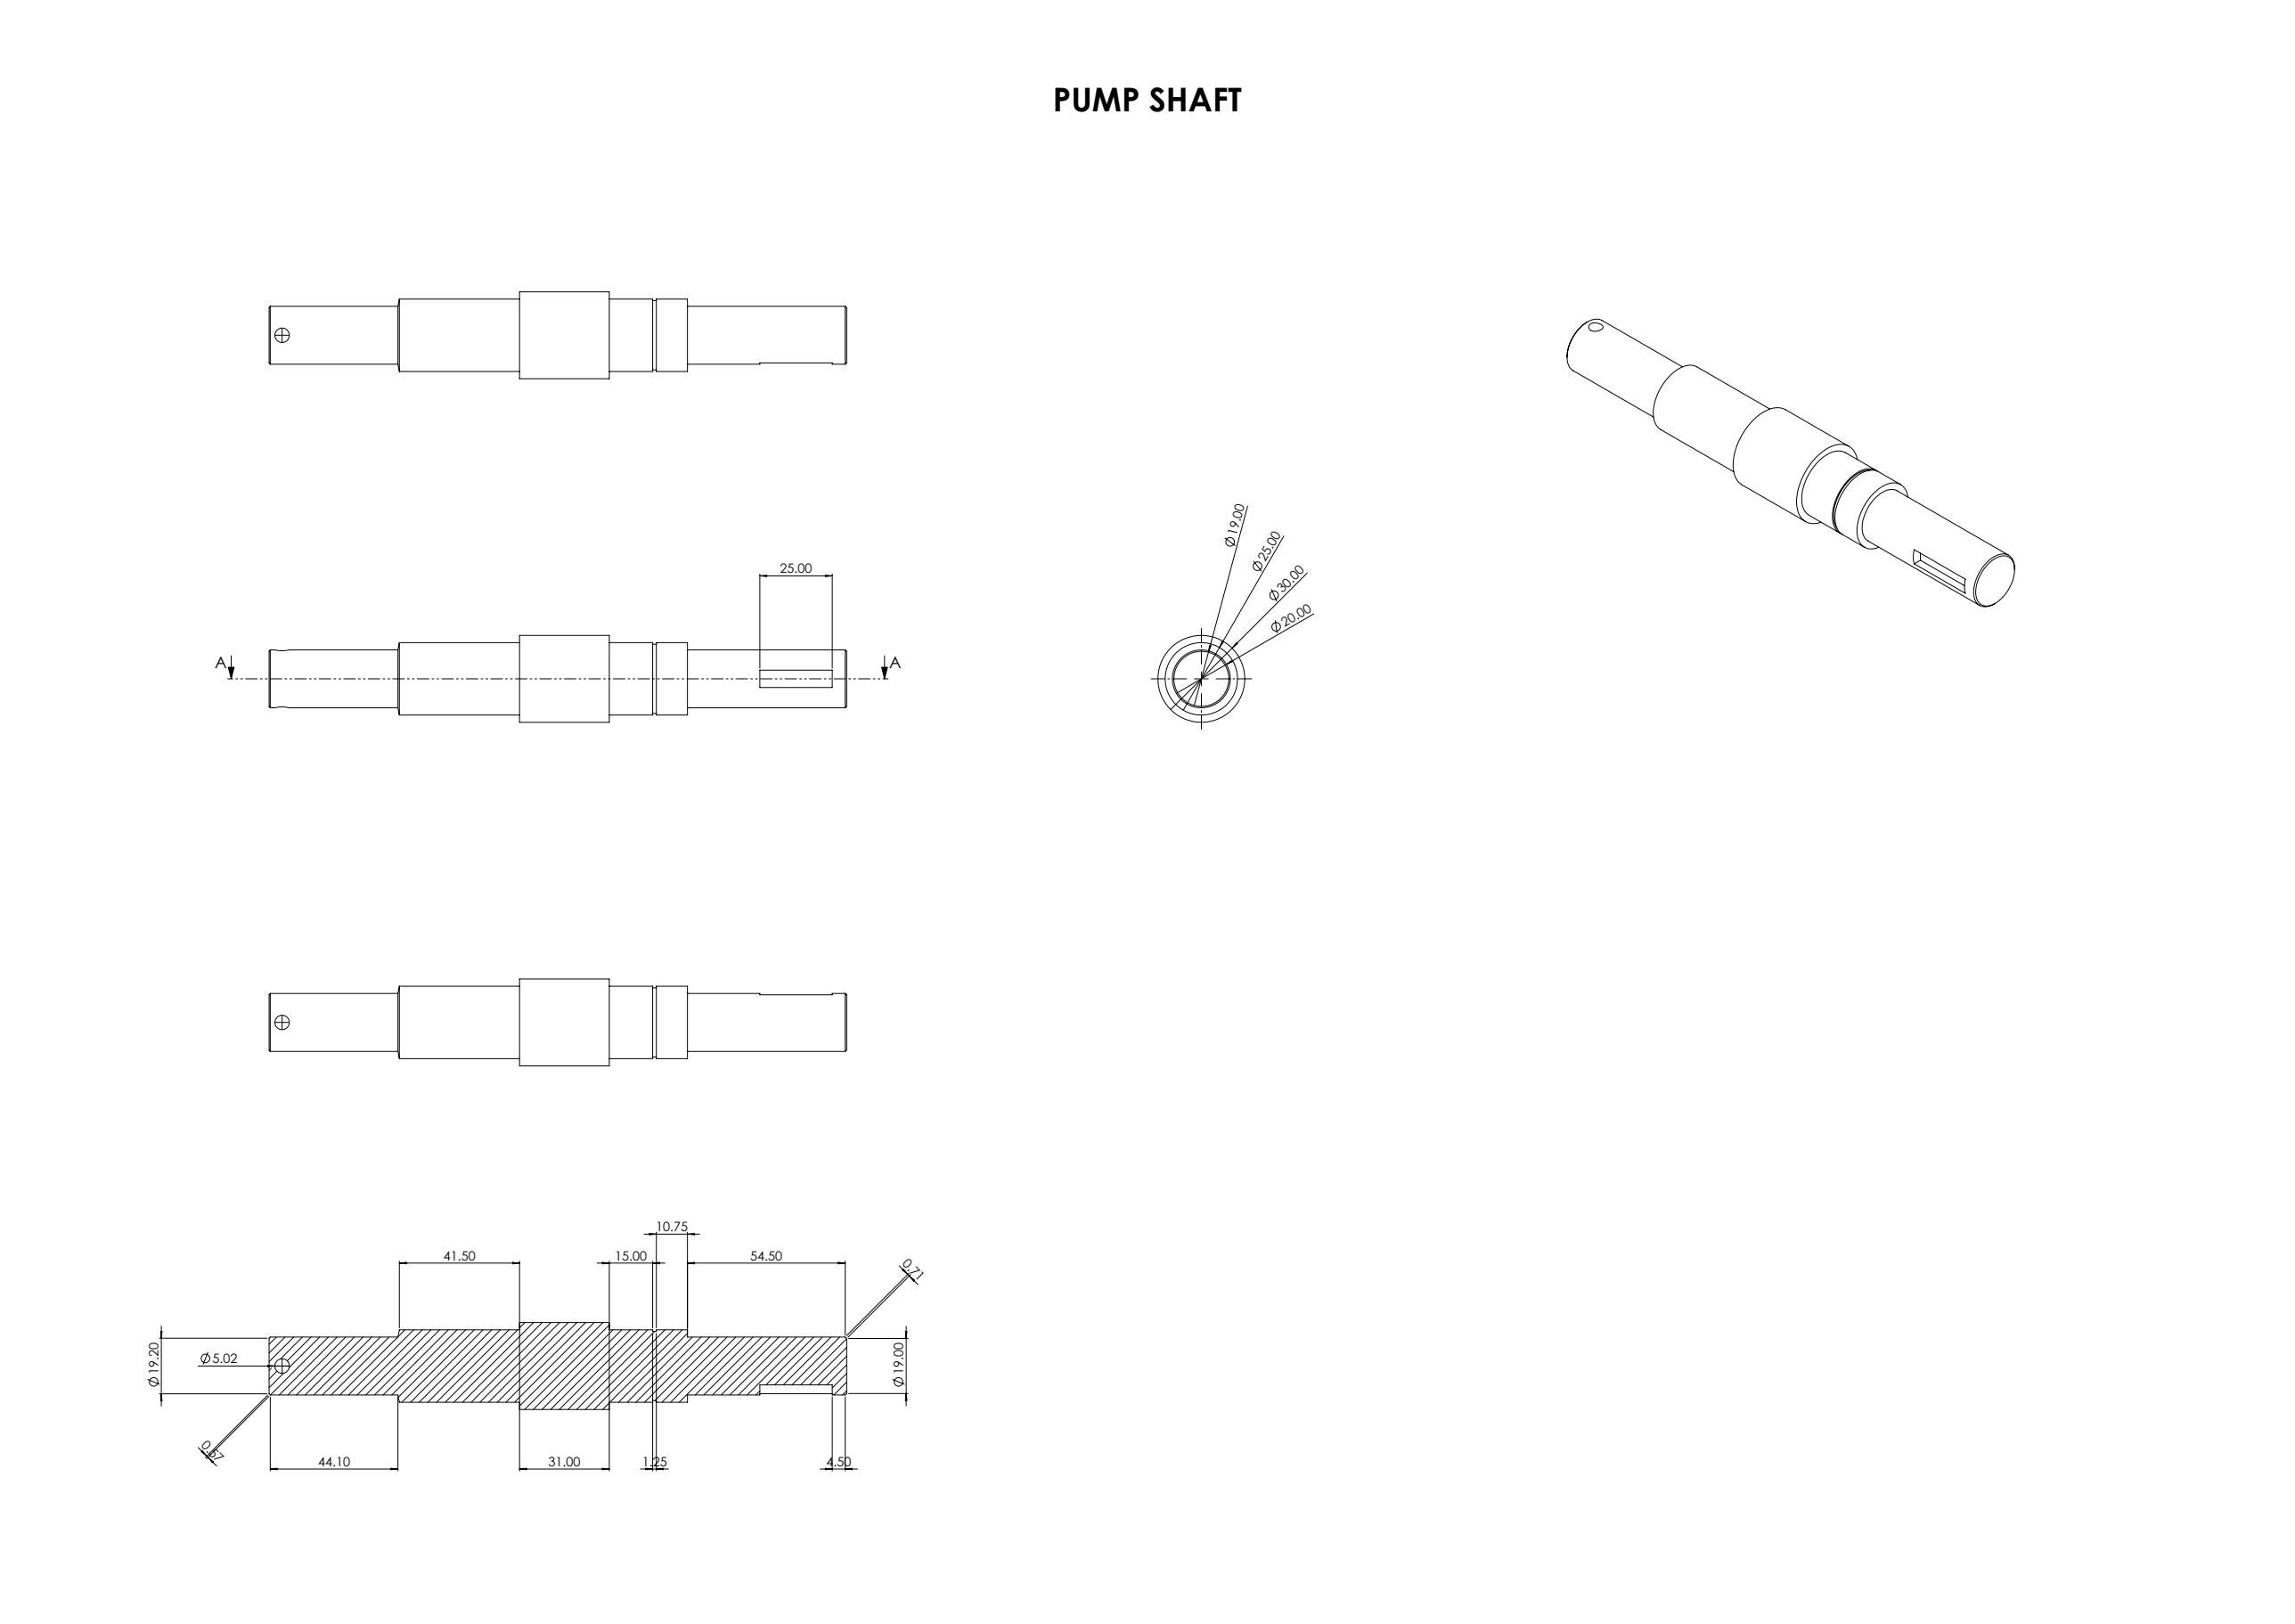
ISO-10303-21;
HEADER;
/* Generated by software containing ST-Developer
 * from STEP Tools, Inc. (www.steptools.com) 
 */

FILE_DESCRIPTION(
/* description */ (''),
/* implementation_level */ '2;1');

FILE_NAME(
/* name */ '05_Pump_Shaft.step',
/* time_stamp */ '2026-10-26T04:15:57-07:00',
/* author */ (''),
/* organization */ (''),
/* preprocessor_version */ 'ST-DEVELOPER v20.2',
/* originating_system */ 'Autodesk Translation Framework v15.15.0.0',
/* authorisation */ '');

FILE_SCHEMA (('AUTOMOTIVE_DESIGN { 1 0 10303 214 3 1 1 }'));
ENDSEC;

DATA;
#10=MECHANICAL_DESIGN_GEOMETRIC_PRESENTATION_REPRESENTATION('',(#456),#55737);
#363=CONICAL_SURFACE('',#29080,9.8,0.785398163397448);
#364=CONICAL_SURFACE('',#29084,11.25,1.37340076694502);
#365=CONICAL_SURFACE('',#29108,9.75,0.785398163397442);
#416=SHAPE_REPRESENTATION_RELATIONSHIP('SRR','None',#55825,#436);
#436=ADVANCED_BREP_SHAPE_REPRESENTATION('',(#476),#55721);
#456=STYLED_ITEM('',(#55991),#476);
#476=MANIFOLD_SOLID_BREP('Body1',#27225);
#683=FACE_BOUND('',#9449,.T.);
#684=FACE_BOUND('',#9453,.T.);
#685=FACE_BOUND('',#9456,.T.);
#686=FACE_BOUND('',#9459,.T.);
#687=FACE_BOUND('',#9462,.T.);
#688=FACE_BOUND('',#9465,.T.);
#689=FACE_BOUND('',#9467,.T.);
#1369=PLANE('',#29070);
#1370=PLANE('',#29072);
#1371=PLANE('',#29073);
#1372=PLANE('',#29074);
#1373=PLANE('',#29076);
#1374=PLANE('',#29078);
#1375=PLANE('',#29088);
#1376=PLANE('',#29092);
#1377=PLANE('',#29096);
#1378=PLANE('',#29100);
#1379=PLANE('',#29104);
#1380=PLANE('',#29110);
#3294=LINE('',#44964,#5665);
#3295=LINE('',#44966,#5666);
#3296=LINE('',#44967,#5667);
#3297=LINE('',#44970,#5668);
#3298=LINE('',#44972,#5669);
#3299=LINE('',#44973,#5670);
#3300=LINE('',#44976,#5671);
#3301=LINE('',#44978,#5672);
#3302=LINE('',#44979,#5673);
#3303=LINE('',#44982,#5674);
#3304=LINE('',#45009,#5675);
#3305=LINE('',#45071,#5676);
#3306=LINE('',#45075,#5677);
#3307=LINE('',#45076,#5678);
#3308=LINE('',#45080,#5679);
#3309=LINE('',#45084,#5680);
#3310=LINE('',#45091,#5681);
#3311=LINE('',#45098,#5682);
#3312=LINE('',#45105,#5683);
#3313=LINE('',#45112,#5684);
#3314=LINE('',#45119,#5685);
#3315=LINE('',#45123,#5686);
#5665=VECTOR('',#34732,10.);
#5666=VECTOR('',#34733,10.);
#5667=VECTOR('',#34734,10.);
#5668=VECTOR('',#34737,10.);
#5669=VECTOR('',#34738,10.);
#5670=VECTOR('',#34739,10.);
#5671=VECTOR('',#34742,10.);
#5672=VECTOR('',#34743,10.);
#5673=VECTOR('',#34744,10.);
#5674=VECTOR('',#34749,10.);
#5675=VECTOR('',#34754,2.51);
#5676=VECTOR('',#34763,9.8);
#5677=VECTOR('',#34768,10.);
#5678=VECTOR('',#34769,10.);
#5679=VECTOR('',#34774,11.25);
#5680=VECTOR('',#34779,12.5);
#5681=VECTOR('',#34788,15.);
#5682=VECTOR('',#34797,12.5);
#5683=VECTOR('',#34806,11.95);
#5684=VECTOR('',#34815,12.5);
#5685=VECTOR('',#34824,10.);
#5686=VECTOR('',#34829,9.75);
#6675=CYLINDRICAL_SURFACE('',#29077,2.51);
#6676=CYLINDRICAL_SURFACE('',#29082,10.);
#6677=CYLINDRICAL_SURFACE('',#29086,12.5);
#6678=CYLINDRICAL_SURFACE('',#29090,15.);
#6679=CYLINDRICAL_SURFACE('',#29094,12.5);
#6680=CYLINDRICAL_SURFACE('',#29098,11.95);
#6681=CYLINDRICAL_SURFACE('',#29102,12.5);
#6682=CYLINDRICAL_SURFACE('',#29106,10.);
#7792=FACE_OUTER_BOUND('',#9440,.T.);
#7793=FACE_OUTER_BOUND('',#9441,.T.);
#7794=FACE_OUTER_BOUND('',#9442,.T.);
#7795=FACE_OUTER_BOUND('',#9443,.T.);
#7796=FACE_OUTER_BOUND('',#9444,.T.);
#7797=FACE_OUTER_BOUND('',#9445,.T.);
#7798=FACE_OUTER_BOUND('',#9446,.T.);
#7799=FACE_OUTER_BOUND('',#9447,.T.);
#7800=FACE_OUTER_BOUND('',#9448,.T.);
#7801=FACE_OUTER_BOUND('',#9450,.T.);
#7802=FACE_OUTER_BOUND('',#9451,.T.);
#7803=FACE_OUTER_BOUND('',#9452,.T.);
#7804=FACE_OUTER_BOUND('',#9454,.T.);
#7805=FACE_OUTER_BOUND('',#9455,.T.);
#7806=FACE_OUTER_BOUND('',#9457,.T.);
#7807=FACE_OUTER_BOUND('',#9458,.T.);
#7808=FACE_OUTER_BOUND('',#9460,.T.);
#7809=FACE_OUTER_BOUND('',#9461,.T.);
#7810=FACE_OUTER_BOUND('',#9463,.T.);
#7811=FACE_OUTER_BOUND('',#9464,.T.);
#7812=FACE_OUTER_BOUND('',#9466,.T.);
#7813=FACE_OUTER_BOUND('',#9468,.T.);
#7814=FACE_OUTER_BOUND('',#9469,.T.);
#9440=EDGE_LOOP('',(#22784,#22785,#22786,#22787));
#9441=EDGE_LOOP('',(#22788,#22789,#22790,#22791));
#9442=EDGE_LOOP('',(#22792,#22793,#22794,#22795));
#9443=EDGE_LOOP('',(#22796,#22797,#22798,#22799));
#9444=EDGE_LOOP('',(#22800,#22801,#22802,#22803));
#9445=EDGE_LOOP('',(#22804,#22805,#22806,#22807,#22808,#22809,#22810));
#9446=EDGE_LOOP('',(#22811));
#9447=EDGE_LOOP('',(#22812,#22813,#22814,#22815));
#9448=EDGE_LOOP('',(#22816,#22817,#22818,#22819,#22820,#22821,#22822,#22823,
#22824));
#9449=EDGE_LOOP('',(#22825,#22826));
#9450=EDGE_LOOP('',(#22827,#22828,#22829,#22830));
#9451=EDGE_LOOP('',(#22831,#22832,#22833,#22834));
#9452=EDGE_LOOP('',(#22835));
#9453=EDGE_LOOP('',(#22836));
#9454=EDGE_LOOP('',(#22837,#22838,#22839,#22840));
#9455=EDGE_LOOP('',(#22841));
#9456=EDGE_LOOP('',(#22842));
#9457=EDGE_LOOP('',(#22843,#22844,#22845,#22846));
#9458=EDGE_LOOP('',(#22847));
#9459=EDGE_LOOP('',(#22848));
#9460=EDGE_LOOP('',(#22849,#22850,#22851,#22852));
#9461=EDGE_LOOP('',(#22853));
#9462=EDGE_LOOP('',(#22854));
#9463=EDGE_LOOP('',(#22855,#22856,#22857,#22858));
#9464=EDGE_LOOP('',(#22859));
#9465=EDGE_LOOP('',(#22860));
#9466=EDGE_LOOP('',(#22861,#22862,#22863,#22864));
#9467=EDGE_LOOP('',(#22865,#22866,#22867,#22868));
#9468=EDGE_LOOP('',(#22869,#22870,#22871,#22872));
#9469=EDGE_LOOP('',(#22873));
#10722=CIRCLE('',#29071,10.);
#10723=CIRCLE('',#29075,10.);
#10724=CIRCLE('',#29079,9.6);
#10725=CIRCLE('',#29081,10.);
#10726=CIRCLE('',#29083,10.);
#10727=CIRCLE('',#29085,12.5);
#10728=CIRCLE('',#29087,12.5);
#10729=CIRCLE('',#29089,15.);
#10730=CIRCLE('',#29091,15.);
#10731=CIRCLE('',#29093,12.5);
#10732=CIRCLE('',#29095,12.5);
#10733=CIRCLE('',#29097,11.95);
#10734=CIRCLE('',#29099,11.95);
#10735=CIRCLE('',#29101,12.5);
#10736=CIRCLE('',#29103,12.5);
#10737=CIRCLE('',#29105,10.);
#10738=CIRCLE('',#29107,10.);
#10739=CIRCLE('',#29109,9.5);
#11189=B_SPLINE_CURVE_WITH_KNOTS('',3,(#44987,#44988,#44989,#44990,#44991,
#44992,#44993,#44994,#44995,#44996),.UNSPECIFIED.,.F.,.F.,(4,2,2,2,4),(0.,
0.0949942193143224,0.189988438628645,0.284969155661888,0.379949872695131),
 .UNSPECIFIED.);
#11190=B_SPLINE_CURVE_WITH_KNOTS('',3,(#44998,#44999,#45000,#45001,#45002,
#45003,#45004,#45005,#45006,#45007),.UNSPECIFIED.,.F.,.F.,(4,2,2,2,4),(1.13984961808539,
1.23483033511864,1.32981105215188,1.4248052714662,1.51979949078052),
 .UNSPECIFIED.);
#11191=B_SPLINE_CURVE_WITH_KNOTS('',3,(#45011,#45012,#45013,#45014,#45015,
#45016,#45017,#45018,#45019,#45020),.UNSPECIFIED.,.F.,.F.,(4,2,2,2,4),(0.,
0.0949942193143224,0.189988438628645,0.284969155661888,0.379949872695131),
 .UNSPECIFIED.);
#11192=B_SPLINE_CURVE_WITH_KNOTS('',3,(#45021,#45022,#45023,#45024,#45025,
#45026,#45027,#45028,#45029,#45030,#45031,#45032,#45033,#45034,#45035,#45036,
#45037,#45038,#45039,#45040,#45041,#45042,#45043,#45044,#45045,#45046),
 .UNSPECIFIED.,.F.,.F.,(4,2,2,2,2,2,2,2,2,2,2,2,4),(0.379949872695131,0.474930589728375,
0.569911306761618,0.66490552607594,0.759899745390262,0.854893964704585,
0.949888184018907,1.04486890105215,1.13984961808539,1.23483033511864,1.32981105215188,
1.4248052714662,1.51979949078053),.UNSPECIFIED.);
#11193=B_SPLINE_CURVE_WITH_KNOTS('',3,(#45047,#45048,#45049,#45050,#45051,
#45052,#45053,#45054,#45055,#45056,#45057,#45058,#45059,#45060,#45061,#45062,
#45063,#45064),.UNSPECIFIED.,.F.,.F.,(4,2,2,2,2,2,2,2,4),(0.379949872695131,
0.474930589728374,0.569911306761618,0.66490552607594,0.759899745390262,
0.854893964704585,0.949888184018907,1.04486890105215,1.13984961808539),
 .UNSPECIFIED.);
#13022=VERTEX_POINT('',#44960);
#13023=VERTEX_POINT('',#44961);
#13024=VERTEX_POINT('',#44963);
#13025=VERTEX_POINT('',#44965);
#13026=VERTEX_POINT('',#44969);
#13027=VERTEX_POINT('',#44971);
#13028=VERTEX_POINT('',#44975);
#13029=VERTEX_POINT('',#44977);
#13030=VERTEX_POINT('',#44985);
#13031=VERTEX_POINT('',#44986);
#13032=VERTEX_POINT('',#44997);
#13033=VERTEX_POINT('',#45008);
#13034=VERTEX_POINT('',#45010);
#13035=VERTEX_POINT('',#45066);
#13036=VERTEX_POINT('',#45069);
#13037=VERTEX_POINT('',#45073);
#13038=VERTEX_POINT('',#45078);
#13039=VERTEX_POINT('',#45082);
#13040=VERTEX_POINT('',#45086);
#13041=VERTEX_POINT('',#45089);
#13042=VERTEX_POINT('',#45093);
#13043=VERTEX_POINT('',#45096);
#13044=VERTEX_POINT('',#45100);
#13045=VERTEX_POINT('',#45103);
#13046=VERTEX_POINT('',#45107);
#13047=VERTEX_POINT('',#45110);
#13048=VERTEX_POINT('',#45114);
#13049=VERTEX_POINT('',#45117);
#13050=VERTEX_POINT('',#45121);
#16396=EDGE_CURVE('',#13022,#13023,#10722,.T.);
#16397=EDGE_CURVE('',#13022,#13024,#3294,.T.);
#16398=EDGE_CURVE('',#13024,#13025,#3295,.T.);
#16399=EDGE_CURVE('',#13023,#13025,#3296,.T.);
#16400=EDGE_CURVE('',#13023,#13026,#3297,.T.);
#16401=EDGE_CURVE('',#13025,#13027,#3298,.T.);
#16402=EDGE_CURVE('',#13026,#13027,#3299,.T.);
#16403=EDGE_CURVE('',#13028,#13022,#3300,.T.);
#16404=EDGE_CURVE('',#13028,#13029,#3301,.T.);
#16405=EDGE_CURVE('',#13029,#13024,#3302,.T.);
#16406=EDGE_CURVE('',#13026,#13028,#10723,.T.);
#16407=EDGE_CURVE('',#13027,#13029,#3303,.T.);
#16408=EDGE_CURVE('',#13030,#13031,#11189,.T.);
#16409=EDGE_CURVE('',#13032,#13030,#11190,.T.);
#16410=EDGE_CURVE('',#13032,#13033,#3304,.T.);
#16411=EDGE_CURVE('',#13034,#13033,#11191,.T.);
#16412=EDGE_CURVE('',#13033,#13034,#11192,.T.);
#16413=EDGE_CURVE('',#13031,#13032,#11193,.T.);
#16414=EDGE_CURVE('',#13035,#13035,#10724,.T.);
#16415=EDGE_CURVE('',#13036,#13036,#10725,.T.);
#16416=EDGE_CURVE('',#13036,#13035,#3305,.T.);
#16417=EDGE_CURVE('',#13037,#13037,#10726,.T.);
#16418=EDGE_CURVE('',#13037,#13031,#3306,.T.);
#16419=EDGE_CURVE('',#13032,#13036,#3307,.T.);
#16420=EDGE_CURVE('',#13038,#13038,#10727,.T.);
#16421=EDGE_CURVE('',#13038,#13037,#3308,.T.);
#16422=EDGE_CURVE('',#13039,#13039,#10728,.T.);
#16423=EDGE_CURVE('',#13039,#13038,#3309,.T.);
#16424=EDGE_CURVE('',#13040,#13040,#10729,.T.);
#16425=EDGE_CURVE('',#13041,#13041,#10730,.T.);
#16426=EDGE_CURVE('',#13041,#13040,#3310,.T.);
#16427=EDGE_CURVE('',#13042,#13042,#10731,.T.);
#16428=EDGE_CURVE('',#13043,#13043,#10732,.T.);
#16429=EDGE_CURVE('',#13043,#13042,#3311,.T.);
#16430=EDGE_CURVE('',#13044,#13044,#10733,.T.);
#16431=EDGE_CURVE('',#13045,#13045,#10734,.T.);
#16432=EDGE_CURVE('',#13045,#13044,#3312,.T.);
#16433=EDGE_CURVE('',#13046,#13046,#10735,.T.);
#16434=EDGE_CURVE('',#13047,#13047,#10736,.T.);
#16435=EDGE_CURVE('',#13047,#13046,#3313,.T.);
#16436=EDGE_CURVE('',#13048,#13048,#10737,.T.);
#16437=EDGE_CURVE('',#13049,#13049,#10738,.T.);
#16438=EDGE_CURVE('',#13049,#13048,#3314,.T.);
#16439=EDGE_CURVE('',#13050,#13050,#10739,.T.);
#16440=EDGE_CURVE('',#13050,#13049,#3315,.T.);
#22784=ORIENTED_EDGE('',*,*,#16396,.F.);
#22785=ORIENTED_EDGE('',*,*,#16397,.T.);
#22786=ORIENTED_EDGE('',*,*,#16398,.T.);
#22787=ORIENTED_EDGE('',*,*,#16399,.F.);
#22788=ORIENTED_EDGE('',*,*,#16400,.F.);
#22789=ORIENTED_EDGE('',*,*,#16399,.T.);
#22790=ORIENTED_EDGE('',*,*,#16401,.T.);
#22791=ORIENTED_EDGE('',*,*,#16402,.F.);
#22792=ORIENTED_EDGE('',*,*,#16403,.F.);
#22793=ORIENTED_EDGE('',*,*,#16404,.T.);
#22794=ORIENTED_EDGE('',*,*,#16405,.T.);
#22795=ORIENTED_EDGE('',*,*,#16397,.F.);
#22796=ORIENTED_EDGE('',*,*,#16406,.F.);
#22797=ORIENTED_EDGE('',*,*,#16402,.T.);
#22798=ORIENTED_EDGE('',*,*,#16407,.T.);
#22799=ORIENTED_EDGE('',*,*,#16404,.F.);
#22800=ORIENTED_EDGE('',*,*,#16398,.F.);
#22801=ORIENTED_EDGE('',*,*,#16405,.F.);
#22802=ORIENTED_EDGE('',*,*,#16407,.F.);
#22803=ORIENTED_EDGE('',*,*,#16401,.F.);
#22804=ORIENTED_EDGE('',*,*,#16408,.F.);
#22805=ORIENTED_EDGE('',*,*,#16409,.F.);
#22806=ORIENTED_EDGE('',*,*,#16410,.T.);
#22807=ORIENTED_EDGE('',*,*,#16411,.F.);
#22808=ORIENTED_EDGE('',*,*,#16412,.F.);
#22809=ORIENTED_EDGE('',*,*,#16410,.F.);
#22810=ORIENTED_EDGE('',*,*,#16413,.F.);
#22811=ORIENTED_EDGE('',*,*,#16414,.F.);
#22812=ORIENTED_EDGE('',*,*,#16415,.F.);
#22813=ORIENTED_EDGE('',*,*,#16416,.T.);
#22814=ORIENTED_EDGE('',*,*,#16414,.T.);
#22815=ORIENTED_EDGE('',*,*,#16416,.F.);
#22816=ORIENTED_EDGE('',*,*,#16417,.F.);
#22817=ORIENTED_EDGE('',*,*,#16418,.T.);
#22818=ORIENTED_EDGE('',*,*,#16413,.T.);
#22819=ORIENTED_EDGE('',*,*,#16419,.T.);
#22820=ORIENTED_EDGE('',*,*,#16415,.T.);
#22821=ORIENTED_EDGE('',*,*,#16419,.F.);
#22822=ORIENTED_EDGE('',*,*,#16409,.T.);
#22823=ORIENTED_EDGE('',*,*,#16408,.T.);
#22824=ORIENTED_EDGE('',*,*,#16418,.F.);
#22825=ORIENTED_EDGE('',*,*,#16411,.T.);
#22826=ORIENTED_EDGE('',*,*,#16412,.T.);
#22827=ORIENTED_EDGE('',*,*,#16420,.F.);
#22828=ORIENTED_EDGE('',*,*,#16421,.T.);
#22829=ORIENTED_EDGE('',*,*,#16417,.T.);
#22830=ORIENTED_EDGE('',*,*,#16421,.F.);
#22831=ORIENTED_EDGE('',*,*,#16422,.F.);
#22832=ORIENTED_EDGE('',*,*,#16423,.T.);
#22833=ORIENTED_EDGE('',*,*,#16420,.T.);
#22834=ORIENTED_EDGE('',*,*,#16423,.F.);
#22835=ORIENTED_EDGE('',*,*,#16424,.F.);
#22836=ORIENTED_EDGE('',*,*,#16422,.T.);
#22837=ORIENTED_EDGE('',*,*,#16425,.F.);
#22838=ORIENTED_EDGE('',*,*,#16426,.T.);
#22839=ORIENTED_EDGE('',*,*,#16424,.T.);
#22840=ORIENTED_EDGE('',*,*,#16426,.F.);
#22841=ORIENTED_EDGE('',*,*,#16425,.T.);
#22842=ORIENTED_EDGE('',*,*,#16427,.F.);
#22843=ORIENTED_EDGE('',*,*,#16428,.F.);
#22844=ORIENTED_EDGE('',*,*,#16429,.T.);
#22845=ORIENTED_EDGE('',*,*,#16427,.T.);
#22846=ORIENTED_EDGE('',*,*,#16429,.F.);
#22847=ORIENTED_EDGE('',*,*,#16428,.T.);
#22848=ORIENTED_EDGE('',*,*,#16430,.F.);
#22849=ORIENTED_EDGE('',*,*,#16431,.F.);
#22850=ORIENTED_EDGE('',*,*,#16432,.T.);
#22851=ORIENTED_EDGE('',*,*,#16430,.T.);
#22852=ORIENTED_EDGE('',*,*,#16432,.F.);
#22853=ORIENTED_EDGE('',*,*,#16433,.F.);
#22854=ORIENTED_EDGE('',*,*,#16431,.T.);
#22855=ORIENTED_EDGE('',*,*,#16434,.F.);
#22856=ORIENTED_EDGE('',*,*,#16435,.T.);
#22857=ORIENTED_EDGE('',*,*,#16433,.T.);
#22858=ORIENTED_EDGE('',*,*,#16435,.F.);
#22859=ORIENTED_EDGE('',*,*,#16434,.T.);
#22860=ORIENTED_EDGE('',*,*,#16436,.F.);
#22861=ORIENTED_EDGE('',*,*,#16437,.F.);
#22862=ORIENTED_EDGE('',*,*,#16438,.T.);
#22863=ORIENTED_EDGE('',*,*,#16436,.T.);
#22864=ORIENTED_EDGE('',*,*,#16438,.F.);
#22865=ORIENTED_EDGE('',*,*,#16406,.T.);
#22866=ORIENTED_EDGE('',*,*,#16403,.T.);
#22867=ORIENTED_EDGE('',*,*,#16396,.T.);
#22868=ORIENTED_EDGE('',*,*,#16400,.T.);
#22869=ORIENTED_EDGE('',*,*,#16439,.F.);
#22870=ORIENTED_EDGE('',*,*,#16440,.T.);
#22871=ORIENTED_EDGE('',*,*,#16437,.T.);
#22872=ORIENTED_EDGE('',*,*,#16440,.F.);
#22873=ORIENTED_EDGE('',*,*,#16439,.T.);
#26616=ADVANCED_FACE('',(#7792),#1369,.F.);
#26617=ADVANCED_FACE('',(#7793),#1370,.F.);
#26618=ADVANCED_FACE('',(#7794),#1371,.F.);
#26619=ADVANCED_FACE('',(#7795),#1372,.F.);
#26620=ADVANCED_FACE('',(#7796),#1373,.F.);
#26621=ADVANCED_FACE('',(#7797),#6675,.F.);
#26622=ADVANCED_FACE('',(#7798),#1374,.T.);
#26623=ADVANCED_FACE('',(#7799),#363,.T.);
#26624=ADVANCED_FACE('',(#7800,#683),#6676,.T.);
#26625=ADVANCED_FACE('',(#7801),#364,.T.);
#26626=ADVANCED_FACE('',(#7802),#6677,.T.);
#26627=ADVANCED_FACE('',(#7803,#684),#1375,.T.);
#26628=ADVANCED_FACE('',(#7804),#6678,.T.);
#26629=ADVANCED_FACE('',(#7805,#685),#1376,.T.);
#26630=ADVANCED_FACE('',(#7806),#6679,.T.);
#26631=ADVANCED_FACE('',(#7807,#686),#1377,.T.);
#26632=ADVANCED_FACE('',(#7808),#6680,.T.);
#26633=ADVANCED_FACE('',(#7809,#687),#1378,.T.);
#26634=ADVANCED_FACE('',(#7810),#6681,.T.);
#26635=ADVANCED_FACE('',(#7811,#688),#1379,.T.);
#26636=ADVANCED_FACE('',(#7812,#689),#6682,.T.);
#26637=ADVANCED_FACE('',(#7813),#365,.T.);
#26638=ADVANCED_FACE('',(#7814),#1380,.T.);
#27225=CLOSED_SHELL('',(#26616,#26617,#26618,#26619,#26620,#26621,#26622,
#26623,#26624,#26625,#26626,#26627,#26628,#26629,#26630,#26631,#26632,#26633,
#26634,#26635,#26636,#26637,#26638));
#29069=AXIS2_PLACEMENT_3D('',#44958,#34726,#34727);
#29070=AXIS2_PLACEMENT_3D('',#44959,#34728,#34729);
#29071=AXIS2_PLACEMENT_3D('',#44962,#34730,#34731);
#29072=AXIS2_PLACEMENT_3D('',#44968,#34735,#34736);
#29073=AXIS2_PLACEMENT_3D('',#44974,#34740,#34741);
#29074=AXIS2_PLACEMENT_3D('',#44980,#34745,#34746);
#29075=AXIS2_PLACEMENT_3D('',#44981,#34747,#34748);
#29076=AXIS2_PLACEMENT_3D('',#44983,#34750,#34751);
#29077=AXIS2_PLACEMENT_3D('',#44984,#34752,#34753);
#29078=AXIS2_PLACEMENT_3D('',#45065,#34755,#34756);
#29079=AXIS2_PLACEMENT_3D('',#45067,#34757,#34758);
#29080=AXIS2_PLACEMENT_3D('',#45068,#34759,#34760);
#29081=AXIS2_PLACEMENT_3D('',#45070,#34761,#34762);
#29082=AXIS2_PLACEMENT_3D('',#45072,#34764,#34765);
#29083=AXIS2_PLACEMENT_3D('',#45074,#34766,#34767);
#29084=AXIS2_PLACEMENT_3D('',#45077,#34770,#34771);
#29085=AXIS2_PLACEMENT_3D('',#45079,#34772,#34773);
#29086=AXIS2_PLACEMENT_3D('',#45081,#34775,#34776);
#29087=AXIS2_PLACEMENT_3D('',#45083,#34777,#34778);
#29088=AXIS2_PLACEMENT_3D('',#45085,#34780,#34781);
#29089=AXIS2_PLACEMENT_3D('',#45087,#34782,#34783);
#29090=AXIS2_PLACEMENT_3D('',#45088,#34784,#34785);
#29091=AXIS2_PLACEMENT_3D('',#45090,#34786,#34787);
#29092=AXIS2_PLACEMENT_3D('',#45092,#34789,#34790);
#29093=AXIS2_PLACEMENT_3D('',#45094,#34791,#34792);
#29094=AXIS2_PLACEMENT_3D('',#45095,#34793,#34794);
#29095=AXIS2_PLACEMENT_3D('',#45097,#34795,#34796);
#29096=AXIS2_PLACEMENT_3D('',#45099,#34798,#34799);
#29097=AXIS2_PLACEMENT_3D('',#45101,#34800,#34801);
#29098=AXIS2_PLACEMENT_3D('',#45102,#34802,#34803);
#29099=AXIS2_PLACEMENT_3D('',#45104,#34804,#34805);
#29100=AXIS2_PLACEMENT_3D('',#45106,#34807,#34808);
#29101=AXIS2_PLACEMENT_3D('',#45108,#34809,#34810);
#29102=AXIS2_PLACEMENT_3D('',#45109,#34811,#34812);
#29103=AXIS2_PLACEMENT_3D('',#45111,#34813,#34814);
#29104=AXIS2_PLACEMENT_3D('',#45113,#34816,#34817);
#29105=AXIS2_PLACEMENT_3D('',#45115,#34818,#34819);
#29106=AXIS2_PLACEMENT_3D('',#45116,#34820,#34821);
#29107=AXIS2_PLACEMENT_3D('',#45118,#34822,#34823);
#29108=AXIS2_PLACEMENT_3D('',#45120,#34825,#34826);
#29109=AXIS2_PLACEMENT_3D('',#45122,#34827,#34828);
#29110=AXIS2_PLACEMENT_3D('',#45124,#34830,#34831);
#34726=DIRECTION('axis',(0.,0.,1.));
#34727=DIRECTION('refdir',(1.,0.,0.));
#34728=DIRECTION('center_axis',(-1.,0.,0.));
#34729=DIRECTION('ref_axis',(0.,1.,0.));
#34730=DIRECTION('center_axis',(-1.,0.,0.));
#34731=DIRECTION('ref_axis',(0.,1.,0.));
#34732=DIRECTION('',(0.,0.,-1.));
#34733=DIRECTION('',(0.,1.,0.));
#34734=DIRECTION('',(0.,0.,-1.));
#34735=DIRECTION('center_axis',(0.,1.,0.));
#34736=DIRECTION('ref_axis',(1.,0.,0.));
#34737=DIRECTION('',(1.,0.,0.));
#34738=DIRECTION('',(1.,0.,0.));
#34739=DIRECTION('',(0.,0.,-1.));
#34740=DIRECTION('center_axis',(0.,-1.,0.));
#34741=DIRECTION('ref_axis',(-1.,0.,0.));
#34742=DIRECTION('',(-1.,0.,0.));
#34743=DIRECTION('',(0.,0.,-1.));
#34744=DIRECTION('',(-1.,0.,0.));
#34745=DIRECTION('center_axis',(1.,0.,0.));
#34746=DIRECTION('ref_axis',(0.,-1.,0.));
#34747=DIRECTION('center_axis',(1.,0.,0.));
#34748=DIRECTION('ref_axis',(0.,1.,0.));
#34749=DIRECTION('',(0.,-1.,0.));
#34750=DIRECTION('center_axis',(0.,0.,-1.));
#34751=DIRECTION('ref_axis',(-1.,0.,0.));
#34752=DIRECTION('center_axis',(0.,1.,0.));
#34753=DIRECTION('ref_axis',(1.,0.,0.));
#34754=DIRECTION('',(0.,1.,0.));
#34755=DIRECTION('center_axis',(-1.,0.,0.));
#34756=DIRECTION('ref_axis',(0.,0.,1.));
#34757=DIRECTION('center_axis',(1.,0.,0.));
#34758=DIRECTION('ref_axis',(0.,0.,-1.));
#34759=DIRECTION('center_axis',(1.,0.,0.));
#34760=DIRECTION('ref_axis',(0.,1.,0.));
#34761=DIRECTION('center_axis',(1.,0.,0.));
#34762=DIRECTION('ref_axis',(0.,0.,-1.));
#34763=DIRECTION('',(-0.707106781186548,0.707106781186548,8.65956056235494E-17));
#34764=DIRECTION('center_axis',(1.,0.,0.));
#34765=DIRECTION('ref_axis',(0.,1.,0.));
#34766=DIRECTION('center_axis',(1.,0.,0.));
#34767=DIRECTION('ref_axis',(0.,0.,-1.));
#34768=DIRECTION('',(-1.,0.,0.));
#34769=DIRECTION('',(-1.,0.,0.));
#34770=DIRECTION('center_axis',(1.,0.,0.));
#34771=DIRECTION('ref_axis',(0.,1.,0.));
#34772=DIRECTION('center_axis',(1.,0.,0.));
#34773=DIRECTION('ref_axis',(0.,0.,-1.));
#34774=DIRECTION('',(-0.196116135138183,0.98058067569092,1.20086498579063E-16));
#34775=DIRECTION('center_axis',(1.,0.,0.));
#34776=DIRECTION('ref_axis',(0.,1.,0.));
#34777=DIRECTION('center_axis',(1.,0.,0.));
#34778=DIRECTION('ref_axis',(0.,0.,-1.));
#34779=DIRECTION('',(-1.,0.,0.));
#34780=DIRECTION('center_axis',(-1.,0.,0.));
#34781=DIRECTION('ref_axis',(0.,0.,1.));
#34782=DIRECTION('center_axis',(1.,0.,0.));
#34783=DIRECTION('ref_axis',(0.,0.,-1.));
#34784=DIRECTION('center_axis',(1.,0.,0.));
#34785=DIRECTION('ref_axis',(0.,1.,0.));
#34786=DIRECTION('center_axis',(1.,0.,0.));
#34787=DIRECTION('ref_axis',(0.,0.,-1.));
#34788=DIRECTION('',(-1.,0.,0.));
#34789=DIRECTION('center_axis',(1.,0.,0.));
#34790=DIRECTION('ref_axis',(0.,0.,-1.));
#34791=DIRECTION('center_axis',(1.,0.,0.));
#34792=DIRECTION('ref_axis',(0.,0.,-1.));
#34793=DIRECTION('center_axis',(1.,0.,0.));
#34794=DIRECTION('ref_axis',(0.,1.,0.));
#34795=DIRECTION('center_axis',(1.,0.,0.));
#34796=DIRECTION('ref_axis',(0.,0.,-1.));
#34797=DIRECTION('',(-1.,0.,0.));
#34798=DIRECTION('center_axis',(1.,0.,0.));
#34799=DIRECTION('ref_axis',(0.,0.,-1.));
#34800=DIRECTION('center_axis',(1.,0.,0.));
#34801=DIRECTION('ref_axis',(0.,0.,-1.));
#34802=DIRECTION('center_axis',(1.,0.,0.));
#34803=DIRECTION('ref_axis',(0.,1.,0.));
#34804=DIRECTION('center_axis',(1.,0.,0.));
#34805=DIRECTION('ref_axis',(0.,0.,-1.));
#34806=DIRECTION('',(-1.,0.,0.));
#34807=DIRECTION('center_axis',(-1.,0.,0.));
#34808=DIRECTION('ref_axis',(0.,0.,1.));
#34809=DIRECTION('center_axis',(1.,0.,0.));
#34810=DIRECTION('ref_axis',(0.,0.,-1.));
#34811=DIRECTION('center_axis',(1.,0.,0.));
#34812=DIRECTION('ref_axis',(0.,1.,0.));
#34813=DIRECTION('center_axis',(1.,0.,0.));
#34814=DIRECTION('ref_axis',(0.,0.,-1.));
#34815=DIRECTION('',(-1.,0.,0.));
#34816=DIRECTION('center_axis',(1.,0.,0.));
#34817=DIRECTION('ref_axis',(0.,0.,-1.));
#34818=DIRECTION('center_axis',(1.,0.,0.));
#34819=DIRECTION('ref_axis',(0.,0.,-1.));
#34820=DIRECTION('center_axis',(1.,0.,0.));
#34821=DIRECTION('ref_axis',(0.,1.,0.));
#34822=DIRECTION('center_axis',(1.,0.,0.));
#34823=DIRECTION('ref_axis',(0.,0.,-1.));
#34824=DIRECTION('',(-1.,0.,0.));
#34825=DIRECTION('center_axis',(-1.,0.,0.));
#34826=DIRECTION('ref_axis',(0.,1.,0.));
#34827=DIRECTION('center_axis',(1.,0.,0.));
#34828=DIRECTION('ref_axis',(0.,0.,-1.));
#34829=DIRECTION('',(-0.707106781186552,-0.707106781186543,-8.65956056235487E-17));
#34830=DIRECTION('center_axis',(1.,0.,0.));
#34831=DIRECTION('ref_axis',(0.,0.,-1.));
#44958=CARTESIAN_POINT('',(0.,0.,0.));
#44959=CARTESIAN_POINT('Origin',(165.,-3.,10.));
#44960=CARTESIAN_POINT('',(165.,-3.,9.53939201416946));
#44961=CARTESIAN_POINT('',(165.,3.,9.53939201416946));
#44962=CARTESIAN_POINT('Origin',(165.,0.,0.));
#44963=CARTESIAN_POINT('',(165.,-3.,6.5));
#44964=CARTESIAN_POINT('',(165.,-3.,10.));
#44965=CARTESIAN_POINT('',(165.,3.,6.5));
#44966=CARTESIAN_POINT('',(165.,3.,6.5));
#44967=CARTESIAN_POINT('',(165.,3.,10.));
#44968=CARTESIAN_POINT('Origin',(165.,3.,10.));
#44969=CARTESIAN_POINT('',(190.,3.,9.53939201416946));
#44970=CARTESIAN_POINT('',(167.25,3.,9.53939201416946));
#44971=CARTESIAN_POINT('',(190.,3.,6.5));
#44972=CARTESIAN_POINT('',(190.,3.,6.5));
#44973=CARTESIAN_POINT('',(190.,3.,10.));
#44974=CARTESIAN_POINT('Origin',(190.,-3.,10.));
#44975=CARTESIAN_POINT('',(190.,-3.,9.53939201416946));
#44976=CARTESIAN_POINT('',(167.25,-3.,9.53939201416946));
#44977=CARTESIAN_POINT('',(190.,-3.,6.5));
#44978=CARTESIAN_POINT('',(190.,-3.,10.));
#44979=CARTESIAN_POINT('',(165.,-3.,6.5));
#44980=CARTESIAN_POINT('Origin',(190.,3.,10.));
#44981=CARTESIAN_POINT('Origin',(190.,0.,0.));
#44982=CARTESIAN_POINT('',(190.,-3.,6.5));
#44983=CARTESIAN_POINT('Origin',(177.5,0.,6.5));
#44984=CARTESIAN_POINT('Origin',(0.,-11.,0.));
#44985=CARTESIAN_POINT('',(1.38777878078145E-16,-9.67987086690727,2.51));
#44986=CARTESIAN_POINT('',(2.51,-10.,-6.81712338612749E-16));
#44987=CARTESIAN_POINT('Ctrl Pts',(-6.93889390390723E-17,-9.67987086690727,
2.51));
#44988=CARTESIAN_POINT('Ctrl Pts',(0.316647397714408,-9.67987086690727,
2.51));
#44989=CARTESIAN_POINT('Ctrl Pts',(0.653424667393654,-9.69702654534655,
2.4464396819459));
#44990=CARTESIAN_POINT('Ctrl Pts',(1.27140541887387,-9.75816738483577,2.18987665098482));
#44991=CARTESIAN_POINT('Ctrl Pts',(1.55273320805174,-9.80118127300772,1.99694283350472));
#44992=CARTESIAN_POINT('Ctrl Pts',(1.99691126398784,-9.8812874714592,1.55276477756863));
#44993=CARTESIAN_POINT('Ctrl Pts',(2.18986969302056,-9.92370211108617,1.27142384596148));
#44994=CARTESIAN_POINT('Ctrl Pts',(2.44645069525432,-9.98345908137755,0.653396472215422));
#44995=CARTESIAN_POINT('Ctrl Pts',(2.51,-10.,0.316602390110811));
#44996=CARTESIAN_POINT('Ctrl Pts',(2.51,-10.,-6.93889390390723E-17));
#44997=CARTESIAN_POINT('',(-2.51,-10.,3.07386346585986E-16));
#44998=CARTESIAN_POINT('Ctrl Pts',(-2.51,-10.,-4.16333634234434E-16));
#44999=CARTESIAN_POINT('Ctrl Pts',(-2.51,-10.,0.31660239011081));
#45000=CARTESIAN_POINT('Ctrl Pts',(-2.44645069525432,-9.98345908137755,
0.65339647221542));
#45001=CARTESIAN_POINT('Ctrl Pts',(-2.18986969302057,-9.92370211108617,
1.27142384596147));
#45002=CARTESIAN_POINT('Ctrl Pts',(-1.99691126398784,-9.8812874714592,1.55276477756863));
#45003=CARTESIAN_POINT('Ctrl Pts',(-1.55273320805175,-9.80118127300772,
1.99694283350472));
#45004=CARTESIAN_POINT('Ctrl Pts',(-1.27140541887387,-9.75816738483577,
2.18987665098481));
#45005=CARTESIAN_POINT('Ctrl Pts',(-0.653424667393656,-9.69702654534655,
2.4464396819459));
#45006=CARTESIAN_POINT('Ctrl Pts',(-0.316647397714409,-9.67987086690727,
2.51));
#45007=CARTESIAN_POINT('Ctrl Pts',(0.,-9.67987086690727,2.51));
#45008=CARTESIAN_POINT('',(-2.51,10.,3.07386346585986E-16));
#45009=CARTESIAN_POINT('',(-2.51,-11.,3.07386346585986E-16));
#45010=CARTESIAN_POINT('',(-6.93889390390723E-17,9.67987086690727,2.51));
#45011=CARTESIAN_POINT('Ctrl Pts',(-6.93889390390723E-17,9.67987086690727,
2.51));
#45012=CARTESIAN_POINT('Ctrl Pts',(-0.316647397714408,9.67987086690727,
2.51));
#45013=CARTESIAN_POINT('Ctrl Pts',(-0.653424667393654,9.69702654534655,
2.4464396819459));
#45014=CARTESIAN_POINT('Ctrl Pts',(-1.27140541887387,9.75816738483577,2.18987665098482));
#45015=CARTESIAN_POINT('Ctrl Pts',(-1.55273320805175,9.80118127300772,1.99694283350472));
#45016=CARTESIAN_POINT('Ctrl Pts',(-1.99691126398784,9.8812874714592,1.55276477756863));
#45017=CARTESIAN_POINT('Ctrl Pts',(-2.18986969302057,9.92370211108617,1.27142384596147));
#45018=CARTESIAN_POINT('Ctrl Pts',(-2.44645069525432,9.98345908137755,0.653396472215421));
#45019=CARTESIAN_POINT('Ctrl Pts',(-2.51,10.,0.31660239011081));
#45020=CARTESIAN_POINT('Ctrl Pts',(-2.51,10.,-3.46944695195361E-16));
#45021=CARTESIAN_POINT('Ctrl Pts',(-2.51,10.,-2.77555756156289E-16));
#45022=CARTESIAN_POINT('Ctrl Pts',(-2.51,10.,-0.316602390110811));
#45023=CARTESIAN_POINT('Ctrl Pts',(-2.44645069525432,9.98345908137755,-0.653396472215422));
#45024=CARTESIAN_POINT('Ctrl Pts',(-2.18986969302056,9.92370211108617,-1.27142384596148));
#45025=CARTESIAN_POINT('Ctrl Pts',(-1.99691126398784,9.8812874714592,-1.55276477756863));
#45026=CARTESIAN_POINT('Ctrl Pts',(-1.55273320805174,9.80118127300772,-1.99694283350472));
#45027=CARTESIAN_POINT('Ctrl Pts',(-1.27140541887387,9.75816738483577,-2.18987665098482));
#45028=CARTESIAN_POINT('Ctrl Pts',(-0.653424667393654,9.69702654534655,
-2.4464396819459));
#45029=CARTESIAN_POINT('Ctrl Pts',(-0.316647397714408,9.67987086690727,
-2.51));
#45030=CARTESIAN_POINT('Ctrl Pts',(0.316647397714408,9.67987086690727,-2.51));
#45031=CARTESIAN_POINT('Ctrl Pts',(0.653424667393654,9.69702654534655,-2.4464396819459));
#45032=CARTESIAN_POINT('Ctrl Pts',(1.27140541887387,9.75816738483577,-2.18987665098482));
#45033=CARTESIAN_POINT('Ctrl Pts',(1.55273320805174,9.80118127300772,-1.99694283350472));
#45034=CARTESIAN_POINT('Ctrl Pts',(1.99691126398784,9.8812874714592,-1.55276477756863));
#45035=CARTESIAN_POINT('Ctrl Pts',(2.18986969302056,9.92370211108617,-1.27142384596148));
#45036=CARTESIAN_POINT('Ctrl Pts',(2.44645069525432,9.98345908137755,-0.653396472215422));
#45037=CARTESIAN_POINT('Ctrl Pts',(2.51,10.,-0.316602390110811));
#45038=CARTESIAN_POINT('Ctrl Pts',(2.51,10.,0.316602390110811));
#45039=CARTESIAN_POINT('Ctrl Pts',(2.44645069525432,9.98345908137755,0.653396472215422));
#45040=CARTESIAN_POINT('Ctrl Pts',(2.18986969302056,9.92370211108617,1.27142384596148));
#45041=CARTESIAN_POINT('Ctrl Pts',(1.99691126398784,9.8812874714592,1.55276477756863));
#45042=CARTESIAN_POINT('Ctrl Pts',(1.55273320805174,9.80118127300772,1.99694283350472));
#45043=CARTESIAN_POINT('Ctrl Pts',(1.27140541887387,9.75816738483577,2.18987665098482));
#45044=CARTESIAN_POINT('Ctrl Pts',(0.653424667393655,9.69702654534655,2.4464396819459));
#45045=CARTESIAN_POINT('Ctrl Pts',(0.316647397714408,9.67987086690727,2.51));
#45046=CARTESIAN_POINT('Ctrl Pts',(-6.93889390390723E-17,9.67987086690727,
2.51));
#45047=CARTESIAN_POINT('Ctrl Pts',(2.51,-10.,0.));
#45048=CARTESIAN_POINT('Ctrl Pts',(2.51,-10.,-0.316602390110811));
#45049=CARTESIAN_POINT('Ctrl Pts',(2.44645069525432,-9.98345908137755,-0.653396472215422));
#45050=CARTESIAN_POINT('Ctrl Pts',(2.18986969302056,-9.92370211108617,-1.27142384596148));
#45051=CARTESIAN_POINT('Ctrl Pts',(1.99691126398784,-9.8812874714592,-1.55276477756863));
#45052=CARTESIAN_POINT('Ctrl Pts',(1.55273320805174,-9.80118127300772,-1.99694283350472));
#45053=CARTESIAN_POINT('Ctrl Pts',(1.27140541887387,-9.75816738483577,-2.18987665098482));
#45054=CARTESIAN_POINT('Ctrl Pts',(0.653424667393654,-9.69702654534655,
-2.4464396819459));
#45055=CARTESIAN_POINT('Ctrl Pts',(0.316647397714408,-9.67987086690727,
-2.51));
#45056=CARTESIAN_POINT('Ctrl Pts',(-0.316647397714408,-9.67987086690727,
-2.51));
#45057=CARTESIAN_POINT('Ctrl Pts',(-0.653424667393654,-9.69702654534655,
-2.4464396819459));
#45058=CARTESIAN_POINT('Ctrl Pts',(-1.27140541887387,-9.75816738483577,
-2.18987665098482));
#45059=CARTESIAN_POINT('Ctrl Pts',(-1.55273320805174,-9.80118127300772,
-1.99694283350472));
#45060=CARTESIAN_POINT('Ctrl Pts',(-1.99691126398784,-9.8812874714592,-1.55276477756863));
#45061=CARTESIAN_POINT('Ctrl Pts',(-2.18986969302057,-9.92370211108617,
-1.27142384596148));
#45062=CARTESIAN_POINT('Ctrl Pts',(-2.44645069525432,-9.98345908137755,
-0.653396472215421));
#45063=CARTESIAN_POINT('Ctrl Pts',(-2.51,-10.,-0.316602390110811));
#45064=CARTESIAN_POINT('Ctrl Pts',(-2.51,-10.,-3.46944695195361E-16));
#45065=CARTESIAN_POINT('Origin',(-4.5,9.6,0.));
#45066=CARTESIAN_POINT('',(-4.49999999999999,-9.6,-1.17566092718146E-15));
#45067=CARTESIAN_POINT('Origin',(-4.49999999999999,0.,0.));
#45068=CARTESIAN_POINT('Origin',(-4.3,0.,0.));
#45069=CARTESIAN_POINT('',(-4.1,-10.,-1.22464679914735E-15));
#45070=CARTESIAN_POINT('Origin',(-4.1,0.,0.));
#45071=CARTESIAN_POINT('',(-4.3,-9.8,-1.20015386316441E-15));
#45072=CARTESIAN_POINT('Origin',(17.95,0.,0.));
#45073=CARTESIAN_POINT('',(40.,-10.,-1.22464679914735E-15));
#45074=CARTESIAN_POINT('Origin',(40.,0.,0.));
#45075=CARTESIAN_POINT('',(17.95,-10.,-1.22464679914735E-15));
#45076=CARTESIAN_POINT('',(17.95,-10.,-1.22464679914735E-15));
#45077=CARTESIAN_POINT('Origin',(40.25,0.,0.));
#45078=CARTESIAN_POINT('',(40.5,-12.5,-1.53080849893419E-15));
#45079=CARTESIAN_POINT('Origin',(40.5,0.,0.));
#45080=CARTESIAN_POINT('',(40.25,-11.25,-1.37772764904077E-15));
#45081=CARTESIAN_POINT('Origin',(61.25,0.,0.));
#45082=CARTESIAN_POINT('',(82.,-12.5,-1.53080849893419E-15));
#45083=CARTESIAN_POINT('Origin',(82.,0.,0.));
#45084=CARTESIAN_POINT('',(61.25,-12.5,-1.53080849893419E-15));
#45085=CARTESIAN_POINT('Origin',(82.,15.,0.));
#45086=CARTESIAN_POINT('',(82.,-15.,-1.83697019872103E-15));
#45087=CARTESIAN_POINT('Origin',(82.,0.,0.));
#45088=CARTESIAN_POINT('Origin',(97.5,0.,0.));
#45089=CARTESIAN_POINT('',(113.,-15.,-1.83697019872103E-15));
#45090=CARTESIAN_POINT('Origin',(113.,0.,0.));
#45091=CARTESIAN_POINT('',(97.5,-15.,-1.83697019872103E-15));
#45092=CARTESIAN_POINT('Origin',(113.,12.5,0.));
#45093=CARTESIAN_POINT('',(113.,-12.5,-1.53080849893419E-15));
#45094=CARTESIAN_POINT('Origin',(113.,0.,0.));
#45095=CARTESIAN_POINT('Origin',(120.5,0.,0.));
#45096=CARTESIAN_POINT('',(128.,-12.5,-1.53080849893419E-15));
#45097=CARTESIAN_POINT('Origin',(128.,0.,0.));
#45098=CARTESIAN_POINT('',(120.5,-12.5,-1.53080849893419E-15));
#45099=CARTESIAN_POINT('Origin',(128.,11.95,0.));
#45100=CARTESIAN_POINT('',(128.,-11.95,-1.46345292498109E-15));
#45101=CARTESIAN_POINT('Origin',(128.,0.,0.));
#45102=CARTESIAN_POINT('Origin',(128.625,0.,0.));
#45103=CARTESIAN_POINT('',(129.25,-11.95,-1.46345292498109E-15));
#45104=CARTESIAN_POINT('Origin',(129.25,0.,0.));
#45105=CARTESIAN_POINT('',(128.625,-11.95,-1.46345292498109E-15));
#45106=CARTESIAN_POINT('Origin',(129.25,12.5,0.));
#45107=CARTESIAN_POINT('',(129.25,-12.5,-1.53080849893419E-15));
#45108=CARTESIAN_POINT('Origin',(129.25,0.,0.));
#45109=CARTESIAN_POINT('Origin',(134.625,0.,0.));
#45110=CARTESIAN_POINT('',(140.,-12.5,-1.53080849893419E-15));
#45111=CARTESIAN_POINT('Origin',(140.,0.,0.));
#45112=CARTESIAN_POINT('',(134.625,-12.5,-1.53080849893419E-15));
#45113=CARTESIAN_POINT('Origin',(140.,10.,0.));
#45114=CARTESIAN_POINT('',(140.,-10.,-1.22464679914735E-15));
#45115=CARTESIAN_POINT('Origin',(140.,0.,0.));
#45116=CARTESIAN_POINT('Origin',(167.25,0.,0.));
#45117=CARTESIAN_POINT('',(194.5,-10.,-1.22464679914735E-15));
#45118=CARTESIAN_POINT('Origin',(194.5,0.,0.));
#45119=CARTESIAN_POINT('',(167.25,-10.,-1.22464679914735E-15));
#45120=CARTESIAN_POINT('Origin',(194.75,0.,0.));
#45121=CARTESIAN_POINT('',(195.,-9.50000000000001,-1.16341445918999E-15));
#45122=CARTESIAN_POINT('Origin',(195.,0.,0.));
#45123=CARTESIAN_POINT('',(194.75,-9.75,-1.19403062916867E-15));
#45124=CARTESIAN_POINT('Origin',(195.,0.,0.));
#55699=UNCERTAINTY_MEASURE_WITH_UNIT(LENGTH_MEASURE(0.01),#55738,
'DISTANCE_ACCURACY_VALUE',
'Maximum model space distance between geometric entities at asserted c
onnectivities');
#55715=UNCERTAINTY_MEASURE_WITH_UNIT(LENGTH_MEASURE(0.01),#55738,
'DISTANCE_ACCURACY_VALUE',
'Maximum model space distance between geometric entities at asserted c
onnectivities');
#55721=(
GEOMETRIC_REPRESENTATION_CONTEXT(3)
GLOBAL_UNCERTAINTY_ASSIGNED_CONTEXT((#55699))
GLOBAL_UNIT_ASSIGNED_CONTEXT((#55738,#55740,#55741))
REPRESENTATION_CONTEXT('','3D')
);
#55737=(
GEOMETRIC_REPRESENTATION_CONTEXT(3)
GLOBAL_UNCERTAINTY_ASSIGNED_CONTEXT((#55715))
GLOBAL_UNIT_ASSIGNED_CONTEXT((#55738,#55740,#55741))
REPRESENTATION_CONTEXT('','3D')
);
#55738=(
LENGTH_UNIT()
NAMED_UNIT(*)
SI_UNIT(.MILLI.,.METRE.)
);
#55740=(
NAMED_UNIT(*)
PLANE_ANGLE_UNIT()
SI_UNIT($,.RADIAN.)
);
#55741=(
NAMED_UNIT(*)
SI_UNIT($,.STERADIAN.)
SOLID_ANGLE_UNIT()
);
#55747=SHAPE_DEFINITION_REPRESENTATION(#55768,#55825);
#55768=PRODUCT_DEFINITION_SHAPE('',$,#55847);
#55825=SHAPE_REPRESENTATION('',(#29069),#55721);
#55841=PRODUCT_DEFINITION_CONTEXT('part definition',#55906,'design');
#55847=PRODUCT_DEFINITION('2026-10-26-00-34-20-668','05_Pump_Shaft',#55868,
#55841);
#55868=PRODUCT_DEFINITION_FORMATION('',$,#55913);
#55906=APPLICATION_CONTEXT(
'Core Data for Automotive Mechanical Design Process');
#55907=PRODUCT_CONTEXT('part definition',#55906,'mechanical');
#55913=PRODUCT('2026-10-26-00-34-20-668','05_Pump_Shaft',$,(#55907));
#55985=COLOUR_RGB('Grey',0.48,0.52,0.57);
#55986=FILL_AREA_STYLE_COLOUR('',#55985);
#55987=FILL_AREA_STYLE('',(#55986));
#55988=SURFACE_STYLE_FILL_AREA(#55987);
#55989=SURFACE_SIDE_STYLE('',(#55988));
#55990=SURFACE_STYLE_USAGE(.BOTH.,#55989);
#55991=PRESENTATION_STYLE_ASSIGNMENT((#55990));
ENDSEC;
END-ISO-10303-21;
